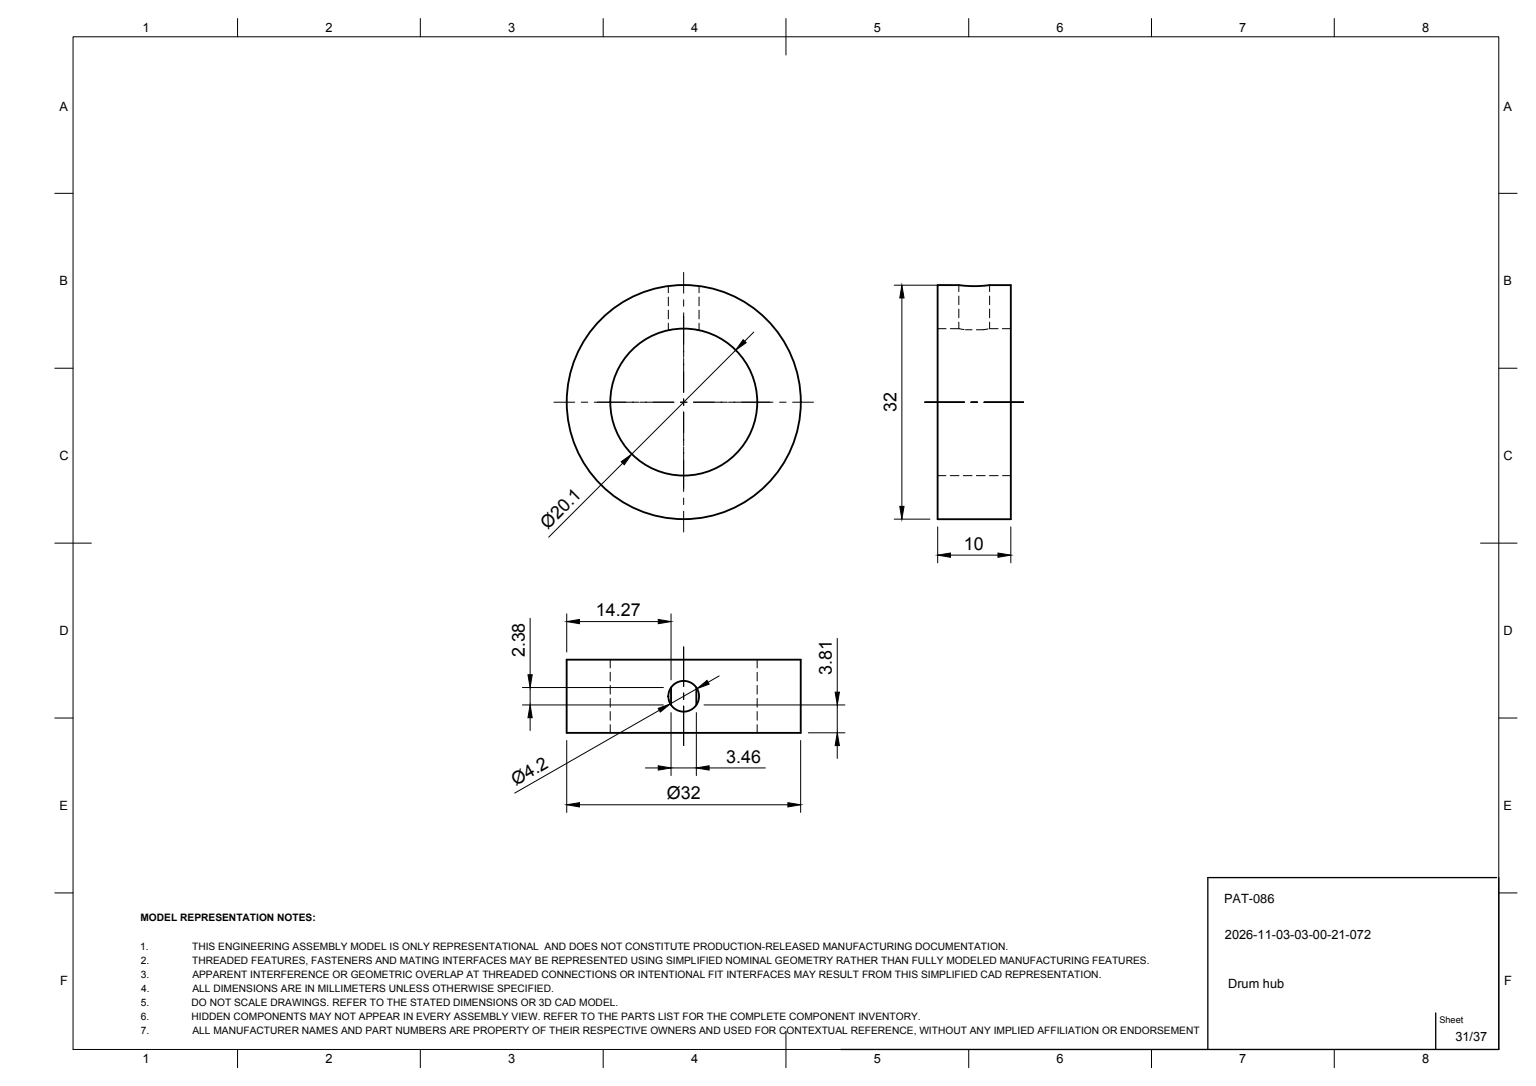
ISO-10303-21;
HEADER;
/* Generated by software containing ST-Developer
 * from STEP Tools, Inc. (www.steptools.com) 
 */

FILE_DESCRIPTION(
/* description */ ('Ratchet and pawl hand winch drum'),
/* implementation_level */ '2;1');

FILE_NAME(
/* name */ 'Drum hub.step',
/* time_stamp */ '2026-10-27T12:42:58-07:00',
/* author */ (''),
/* organization */ (''),
/* preprocessor_version */ 'ST-DEVELOPER v20.2',
/* originating_system */ 'Autodesk Translation Framework v15.17.0.0',
/* authorisation */ '');

FILE_SCHEMA (('AUTOMOTIVE_DESIGN { 1 0 10303 214 3 1 1 }'));
ENDSEC;

DATA;
#10=MECHANICAL_DESIGN_GEOMETRIC_PRESENTATION_REPRESENTATION('',(#415),#11801);
#305=B_SPLINE_CURVE_WITH_KNOTS('',3,(#10818,#10819,#10820,#10821,#10822,
#10823,#10824,#10825,#10826,#10827,#10828,#10829,#10830,#10831),
 .UNSPECIFIED.,.F.,.F.,(4,2,2,2,2,2,4),(0.756005737987019,0.793568827564647,
0.872922520054201,0.952276212543756,1.03162990503331,1.11098359752287,1.14854668710049),
 .UNSPECIFIED.);
#306=B_SPLINE_CURVE_WITH_KNOTS('',3,(#10837,#10838,#10839,#10840,#10841,
#10842,#10843,#10844,#10845,#10846,#10847,#10848,#10849,#10850,#10851,#10852,
#10853,#10854),.UNSPECIFIED.,.F.,.F.,(4,2,2,2,2,2,2,2,4),(0.,0.0792028026112439,
0.158405605222488,0.237607602356377,0.316809599490267,0.396011596624156,
0.475213593758045,0.554416396369289,0.633619198980533),.UNSPECIFIED.);
#307=B_SPLINE_CURVE_WITH_KNOTS('',3,(#10855,#10856,#10857,#10858,#10859,
#10860,#10861,#10862,#10863,#10864,#10865,#10866,#10867,#10868,#10869,#10870,
#10871,#10872),.UNSPECIFIED.,.F.,.F.,(4,2,2,2,2,2,2,2,4),(0.633619198980533,
0.712822001591777,0.792024804203021,0.87122680133691,0.950428798470799,
1.02963079560469,1.10883279273858,1.18803559534982,1.26723839796107),
 .UNSPECIFIED.);
#308=B_SPLINE_CURVE_WITH_KNOTS('',3,(#10875,#10876,#10877,#10878,#10879,
#10880,#10881,#10882,#10883,#10884,#10885,#10886,#10887,#10888),
 .UNSPECIFIED.,.F.,.F.,(4,2,2,2,2,2,4),(0.121154929624516,0.158718019202143,
0.238071711691697,0.317425404181252,0.396779096670807,0.476132789160362,
0.513695878737988),.UNSPECIFIED.);
#346=SHAPE_REPRESENTATION_RELATIONSHIP('SRR','None',#11974,#380);
#380=ADVANCED_BREP_SHAPE_REPRESENTATION('',(#448),#11791);
#415=STYLED_ITEM('',(#12199),#448);
#448=MANIFOLD_SOLID_BREP('Body1',#6294);
#576=FACE_BOUND('',#1548,.T.);
#577=FACE_BOUND('',#1550,.T.);
#578=FACE_BOUND('',#1552,.T.);
#579=FACE_BOUND('',#1554,.T.);
#740=PLANE('',#7105);
#741=PLANE('',#7110);
#742=PLANE('',#7117);
#743=PLANE('',#7118);
#1068=FACE_OUTER_BOUND('',#1544,.T.);
#1069=FACE_OUTER_BOUND('',#1545,.T.);
#1070=FACE_OUTER_BOUND('',#1546,.T.);
#1071=FACE_OUTER_BOUND('',#1547,.T.);
#1072=FACE_OUTER_BOUND('',#1549,.T.);
#1073=FACE_OUTER_BOUND('',#1551,.T.);
#1074=FACE_OUTER_BOUND('',#1553,.T.);
#1544=EDGE_LOOP('',(#5195,#5196));
#1545=EDGE_LOOP('',(#5197,#5198,#5199,#5200,#5201,#5202,#5203,#5204,#5205));
#1546=EDGE_LOOP('',(#5206,#5207,#5208));
#1547=EDGE_LOOP('',(#5209,#5210,#5211,#5212));
#1548=EDGE_LOOP('',(#5213,#5214,#5215,#5216));
#1549=EDGE_LOOP('',(#5217,#5218,#5219,#5220));
#1550=EDGE_LOOP('',(#5221,#5222));
#1551=EDGE_LOOP('',(#5223));
#1552=EDGE_LOOP('',(#5224));
#1553=EDGE_LOOP('',(#5225));
#1554=EDGE_LOOP('',(#5226));
#1973=LINE('',#10814,#2484);
#1974=LINE('',#10835,#2485);
#1975=LINE('',#10890,#2486);
#1976=LINE('',#10895,#2487);
#1977=LINE('',#10901,#2488);
#2484=VECTOR('',#8488,1.);
#2485=VECTOR('',#8495,0.21);
#2486=VECTOR('',#8500,1.);
#2487=VECTOR('',#8505,1.005);
#2488=VECTOR('',#8512,1.6);
#2885=CIRCLE('',#7106,0.21);
#2886=CIRCLE('',#7108,0.21);
#2887=CIRCLE('',#7109,0.21);
#2888=CIRCLE('',#7112,1.005);
#2889=CIRCLE('',#7113,1.005);
#2890=CIRCLE('',#7115,1.6);
#2891=CIRCLE('',#7116,1.6);
#3264=VERTEX_POINT('',#10812);
#3265=VERTEX_POINT('',#10813);
#3266=VERTEX_POINT('',#10817);
#3267=VERTEX_POINT('',#10832);
#3268=VERTEX_POINT('',#10834);
#3269=VERTEX_POINT('',#10836);
#3270=VERTEX_POINT('',#10873);
#3271=VERTEX_POINT('',#10892);
#3272=VERTEX_POINT('',#10894);
#3273=VERTEX_POINT('',#10898);
#3274=VERTEX_POINT('',#10900);
#3941=EDGE_CURVE('',#3264,#3265,#1973,.T.);
#3942=EDGE_CURVE('',#3264,#3265,#2885,.T.);
#3943=EDGE_CURVE('',#3266,#3264,#305,.T.);
#3944=EDGE_CURVE('',#3267,#3266,#2886,.T.);
#3945=EDGE_CURVE('',#3267,#3268,#1974,.T.);
#3946=EDGE_CURVE('',#3269,#3268,#306,.T.);
#3947=EDGE_CURVE('',#3268,#3269,#307,.T.);
#3948=EDGE_CURVE('',#3270,#3267,#2887,.T.);
#3949=EDGE_CURVE('',#3265,#3270,#308,.T.);
#3950=EDGE_CURVE('',#3270,#3266,#1975,.T.);
#3951=EDGE_CURVE('',#3271,#3271,#2888,.T.);
#3952=EDGE_CURVE('',#3271,#3272,#1976,.T.);
#3953=EDGE_CURVE('',#3272,#3272,#2889,.T.);
#3954=EDGE_CURVE('',#3273,#3273,#2890,.T.);
#3955=EDGE_CURVE('',#3273,#3274,#1977,.T.);
#3956=EDGE_CURVE('',#3274,#3274,#2891,.T.);
#5195=ORIENTED_EDGE('',*,*,#3941,.F.);
#5196=ORIENTED_EDGE('',*,*,#3942,.T.);
#5197=ORIENTED_EDGE('',*,*,#3943,.F.);
#5198=ORIENTED_EDGE('',*,*,#3944,.F.);
#5199=ORIENTED_EDGE('',*,*,#3945,.T.);
#5200=ORIENTED_EDGE('',*,*,#3946,.F.);
#5201=ORIENTED_EDGE('',*,*,#3947,.F.);
#5202=ORIENTED_EDGE('',*,*,#3945,.F.);
#5203=ORIENTED_EDGE('',*,*,#3948,.F.);
#5204=ORIENTED_EDGE('',*,*,#3949,.F.);
#5205=ORIENTED_EDGE('',*,*,#3942,.F.);
#5206=ORIENTED_EDGE('',*,*,#3950,.F.);
#5207=ORIENTED_EDGE('',*,*,#3948,.T.);
#5208=ORIENTED_EDGE('',*,*,#3944,.T.);
#5209=ORIENTED_EDGE('',*,*,#3951,.F.);
#5210=ORIENTED_EDGE('',*,*,#3952,.T.);
#5211=ORIENTED_EDGE('',*,*,#3953,.T.);
#5212=ORIENTED_EDGE('',*,*,#3952,.F.);
#5213=ORIENTED_EDGE('',*,*,#3949,.T.);
#5214=ORIENTED_EDGE('',*,*,#3950,.T.);
#5215=ORIENTED_EDGE('',*,*,#3943,.T.);
#5216=ORIENTED_EDGE('',*,*,#3941,.T.);
#5217=ORIENTED_EDGE('',*,*,#3954,.F.);
#5218=ORIENTED_EDGE('',*,*,#3955,.T.);
#5219=ORIENTED_EDGE('',*,*,#3956,.T.);
#5220=ORIENTED_EDGE('',*,*,#3955,.F.);
#5221=ORIENTED_EDGE('',*,*,#3946,.T.);
#5222=ORIENTED_EDGE('',*,*,#3947,.T.);
#5223=ORIENTED_EDGE('',*,*,#3954,.T.);
#5224=ORIENTED_EDGE('',*,*,#3951,.T.);
#5225=ORIENTED_EDGE('',*,*,#3956,.F.);
#5226=ORIENTED_EDGE('',*,*,#3953,.F.);
#5888=CYLINDRICAL_SURFACE('',#7107,0.21);
#5889=CYLINDRICAL_SURFACE('',#7111,1.005);
#5890=CYLINDRICAL_SURFACE('',#7114,1.6);
#6138=ADVANCED_FACE('',(#1068),#740,.T.);
#6139=ADVANCED_FACE('',(#1069),#5888,.F.);
#6140=ADVANCED_FACE('',(#1070),#741,.T.);
#6141=ADVANCED_FACE('',(#1071,#576),#5889,.F.);
#6142=ADVANCED_FACE('',(#1072,#577),#5890,.T.);
#6143=ADVANCED_FACE('',(#1073,#578),#742,.T.);
#6144=ADVANCED_FACE('',(#1074,#579),#743,.F.);
#6294=CLOSED_SHELL('',(#6138,#6139,#6140,#6141,#6142,#6143,#6144));
#7104=AXIS2_PLACEMENT_3D('',#10810,#8484,#8485);
#7105=AXIS2_PLACEMENT_3D('',#10811,#8486,#8487);
#7106=AXIS2_PLACEMENT_3D('',#10815,#8489,#8490);
#7107=AXIS2_PLACEMENT_3D('',#10816,#8491,#8492);
#7108=AXIS2_PLACEMENT_3D('',#10833,#8493,#8494);
#7109=AXIS2_PLACEMENT_3D('',#10874,#8496,#8497);
#7110=AXIS2_PLACEMENT_3D('',#10889,#8498,#8499);
#7111=AXIS2_PLACEMENT_3D('',#10891,#8501,#8502);
#7112=AXIS2_PLACEMENT_3D('',#10893,#8503,#8504);
#7113=AXIS2_PLACEMENT_3D('',#10896,#8506,#8507);
#7114=AXIS2_PLACEMENT_3D('',#10897,#8508,#8509);
#7115=AXIS2_PLACEMENT_3D('',#10899,#8510,#8511);
#7116=AXIS2_PLACEMENT_3D('',#10902,#8513,#8514);
#7117=AXIS2_PLACEMENT_3D('',#10903,#8515,#8516);
#7118=AXIS2_PLACEMENT_3D('',#10904,#8517,#8518);
#8484=DIRECTION('axis',(0.,0.,1.));
#8485=DIRECTION('refdir',(1.,0.,0.));
#8486=DIRECTION('center_axis',(0.,0.,1.));
#8487=DIRECTION('ref_axis',(1.,0.,0.));
#8488=DIRECTION('',(0.,1.,0.));
#8489=DIRECTION('center_axis',(0.,0.,1.));
#8490=DIRECTION('ref_axis',(1.,0.,0.));
#8491=DIRECTION('center_axis',(0.,0.,1.));
#8492=DIRECTION('ref_axis',(1.,0.,0.));
#8493=DIRECTION('center_axis',(0.,0.,1.));
#8494=DIRECTION('ref_axis',(1.,0.,0.));
#8495=DIRECTION('',(0.,0.,1.));
#8496=DIRECTION('center_axis',(0.,0.,1.));
#8497=DIRECTION('ref_axis',(1.,0.,0.));
#8498=DIRECTION('center_axis',(0.,0.,1.));
#8499=DIRECTION('ref_axis',(1.,0.,0.));
#8500=DIRECTION('',(0.,-1.,0.));
#8501=DIRECTION('center_axis',(0.,1.,0.));
#8502=DIRECTION('ref_axis',(1.,0.,0.));
#8503=DIRECTION('center_axis',(0.,-1.,0.));
#8504=DIRECTION('ref_axis',(1.,0.,0.));
#8505=DIRECTION('',(0.,-1.,0.));
#8506=DIRECTION('center_axis',(0.,-1.,0.));
#8507=DIRECTION('ref_axis',(1.,0.,0.));
#8508=DIRECTION('center_axis',(0.,1.,0.));
#8509=DIRECTION('ref_axis',(1.,0.,0.));
#8510=DIRECTION('center_axis',(0.,1.,0.));
#8511=DIRECTION('ref_axis',(1.,0.,0.));
#8512=DIRECTION('',(0.,-1.,0.));
#8513=DIRECTION('center_axis',(0.,1.,0.));
#8514=DIRECTION('ref_axis',(1.,0.,0.));
#8515=DIRECTION('center_axis',(0.,1.,0.));
#8516=DIRECTION('ref_axis',(1.,0.,0.));
#8517=DIRECTION('center_axis',(0.,1.,0.));
#8518=DIRECTION('ref_axis',(1.,0.,0.));
#10810=CARTESIAN_POINT('',(0.,0.,0.));
#10811=CARTESIAN_POINT('Origin',(0.,3.5,7.52));
#10812=CARTESIAN_POINT('',(0.172988438920056,3.38094119100209,7.52));
#10813=CARTESIAN_POINT('',(0.172988438920056,3.61905880899792,7.52));
#10814=CARTESIAN_POINT('',(0.172988438920056,3.,7.52));
#10815=CARTESIAN_POINT('Origin',(0.,3.5,7.52));
#10816=CARTESIAN_POINT('Origin',(0.,3.5,7.52));
#10817=CARTESIAN_POINT('',(-0.172988438920056,3.38094119100209,7.52));
#10818=CARTESIAN_POINT('Ctrl Pts',(-0.172988438920056,3.38094119100209,
7.52));
#10819=CARTESIAN_POINT('Ctrl Pts',(-0.165594865311315,3.37019857760471,
7.52129192197638));
#10820=CARTESIAN_POINT('Ctrl Pts',(-0.157297138725606,3.36031229062726,
7.52265394943905));
#10821=CARTESIAN_POINT('Ctrl Pts',(-0.129892073845076,3.33290722574673,
7.5267480843909));
#10822=CARTESIAN_POINT('Ctrl Pts',(-0.106330167759285,3.31675794366705,
7.52969589327638));
#10823=CARTESIAN_POINT('Ctrl Pts',(-0.0546129046324106,3.29530220603509,
7.53385029472357));
#10824=CARTESIAN_POINT('Ctrl Pts',(-0.0264512308298517,3.29,7.535));
#10825=CARTESIAN_POINT('Ctrl Pts',(0.0264512308298516,3.29,7.535));
#10826=CARTESIAN_POINT('Ctrl Pts',(0.0546129046324105,3.29530220603509,
7.53385029472357));
#10827=CARTESIAN_POINT('Ctrl Pts',(0.106330167759284,3.31675794366705,7.52969589327638));
#10828=CARTESIAN_POINT('Ctrl Pts',(0.129892073845076,3.33290722574673,7.5267480843909));
#10829=CARTESIAN_POINT('Ctrl Pts',(0.157297138725606,3.36031229062726,7.52265394943905));
#10830=CARTESIAN_POINT('Ctrl Pts',(0.165594865311315,3.37019857760471,7.52129192197638));
#10831=CARTESIAN_POINT('Ctrl Pts',(0.172988438920056,3.38094119100209,7.52));
#10832=CARTESIAN_POINT('',(-0.21,3.5,7.52));
#10833=CARTESIAN_POINT('Origin',(0.,3.5,7.52));
#10834=CARTESIAN_POINT('',(-0.21,3.5,8.11615888233178));
#10835=CARTESIAN_POINT('',(-0.21,3.5,7.52));
#10836=CARTESIAN_POINT('',(0.21,3.5,8.11615888233178));
#10837=CARTESIAN_POINT('Ctrl Pts',(0.21,3.5,8.11615888233178));
#10838=CARTESIAN_POINT('Ctrl Pts',(0.21,3.47359906579625,8.11615888233178));
#10839=CARTESIAN_POINT('Ctrl Pts',(0.20471752266132,3.44545944463489,8.11688606295397));
#10840=CARTESIAN_POINT('Ctrl Pts',(0.183276841782292,3.3937289476995,8.11950502964782));
#10841=CARTESIAN_POINT('Ctrl Pts',(0.167120287247804,3.37013543914945,8.12135816887013));
#10842=CARTESIAN_POINT('Ctrl Pts',(0.129864750292352,3.332879902194,8.12483075953278));
#10843=CARTESIAN_POINT('Ctrl Pts',(0.106271159541076,3.31672319916877,8.12667690933009));
#10844=CARTESIAN_POINT('Ctrl Pts',(0.0545403836274688,3.2952824096556,8.12927985626981));
#10845=CARTESIAN_POINT('Ctrl Pts',(0.0264006657112965,3.29,8.13));
#10846=CARTESIAN_POINT('Ctrl Pts',(-0.0264006657112964,3.29,8.13));
#10847=CARTESIAN_POINT('Ctrl Pts',(-0.0545403836274688,3.2952824096556,
8.12927985626981));
#10848=CARTESIAN_POINT('Ctrl Pts',(-0.106271159541076,3.31672319916877,
8.12667690933009));
#10849=CARTESIAN_POINT('Ctrl Pts',(-0.129864750292352,3.332879902194,8.12483075953278));
#10850=CARTESIAN_POINT('Ctrl Pts',(-0.167120287247804,3.37013543914945,
8.12135816887013));
#10851=CARTESIAN_POINT('Ctrl Pts',(-0.183276841782292,3.3937289476995,8.11950502964782));
#10852=CARTESIAN_POINT('Ctrl Pts',(-0.20471752266132,3.44545944463489,8.11688606295397));
#10853=CARTESIAN_POINT('Ctrl Pts',(-0.21,3.47359906579625,8.11615888233178));
#10854=CARTESIAN_POINT('Ctrl Pts',(-0.21,3.5,8.11615888233178));
#10855=CARTESIAN_POINT('Ctrl Pts',(-0.21,3.5,8.11615888233178));
#10856=CARTESIAN_POINT('Ctrl Pts',(-0.21,3.52640093420375,8.11615888233178));
#10857=CARTESIAN_POINT('Ctrl Pts',(-0.20471752266132,3.55454055536511,8.11688606295397));
#10858=CARTESIAN_POINT('Ctrl Pts',(-0.183276841782292,3.6062710523005,8.11950502964782));
#10859=CARTESIAN_POINT('Ctrl Pts',(-0.167120287247804,3.62986456085055,
8.12135816887013));
#10860=CARTESIAN_POINT('Ctrl Pts',(-0.129864750292352,3.667120097806,8.12483075953278));
#10861=CARTESIAN_POINT('Ctrl Pts',(-0.106271159541076,3.68327680083123,
8.12667690933009));
#10862=CARTESIAN_POINT('Ctrl Pts',(-0.0545403836274688,3.7047175903444,
8.12927985626981));
#10863=CARTESIAN_POINT('Ctrl Pts',(-0.0264006657112965,3.71,8.13));
#10864=CARTESIAN_POINT('Ctrl Pts',(0.0264006657112965,3.71,8.13));
#10865=CARTESIAN_POINT('Ctrl Pts',(0.0545403836274689,3.7047175903444,8.12927985626981));
#10866=CARTESIAN_POINT('Ctrl Pts',(0.106271159541076,3.68327680083123,8.12667690933009));
#10867=CARTESIAN_POINT('Ctrl Pts',(0.129864750292352,3.667120097806,8.12483075953278));
#10868=CARTESIAN_POINT('Ctrl Pts',(0.167120287247804,3.62986456085055,8.12135816887013));
#10869=CARTESIAN_POINT('Ctrl Pts',(0.183276841782292,3.6062710523005,8.11950502964782));
#10870=CARTESIAN_POINT('Ctrl Pts',(0.20471752266132,3.55454055536511,8.11688606295397));
#10871=CARTESIAN_POINT('Ctrl Pts',(0.21,3.52640093420375,8.11615888233178));
#10872=CARTESIAN_POINT('Ctrl Pts',(0.21,3.5,8.11615888233178));
#10873=CARTESIAN_POINT('',(-0.172988438920056,3.61905880899792,7.52));
#10874=CARTESIAN_POINT('Origin',(0.,3.5,7.52));
#10875=CARTESIAN_POINT('Ctrl Pts',(0.172988438920056,3.61905880899792,7.52));
#10876=CARTESIAN_POINT('Ctrl Pts',(0.165594865311314,3.62980142239529,7.52129192197638));
#10877=CARTESIAN_POINT('Ctrl Pts',(0.157297138725606,3.63968770937274,7.52265394943905));
#10878=CARTESIAN_POINT('Ctrl Pts',(0.129892073845076,3.66709277425327,7.5267480843909));
#10879=CARTESIAN_POINT('Ctrl Pts',(0.106330167759284,3.68324205633295,7.52969589327638));
#10880=CARTESIAN_POINT('Ctrl Pts',(0.0546129046324106,3.70469779396491,
7.53385029472357));
#10881=CARTESIAN_POINT('Ctrl Pts',(0.0264512308298516,3.71,7.535));
#10882=CARTESIAN_POINT('Ctrl Pts',(-0.0264512308298516,3.71,7.535));
#10883=CARTESIAN_POINT('Ctrl Pts',(-0.0546129046324105,3.70469779396491,
7.53385029472357));
#10884=CARTESIAN_POINT('Ctrl Pts',(-0.106330167759284,3.68324205633295,
7.52969589327638));
#10885=CARTESIAN_POINT('Ctrl Pts',(-0.129892073845076,3.66709277425327,
7.5267480843909));
#10886=CARTESIAN_POINT('Ctrl Pts',(-0.157297138725606,3.63968770937274,
7.52265394943905));
#10887=CARTESIAN_POINT('Ctrl Pts',(-0.165594865311314,3.62980142239529,
7.52129192197638));
#10888=CARTESIAN_POINT('Ctrl Pts',(-0.172988438920056,3.61905880899792,
7.52));
#10889=CARTESIAN_POINT('Origin',(0.,3.5,7.52));
#10890=CARTESIAN_POINT('',(-0.172988438920056,3.,7.52));
#10891=CARTESIAN_POINT('Origin',(0.,3.,6.53));
#10892=CARTESIAN_POINT('',(-1.005,4.,6.53));
#10893=CARTESIAN_POINT('Origin',(0.,4.,6.53));
#10894=CARTESIAN_POINT('',(-1.005,3.,6.53));
#10895=CARTESIAN_POINT('',(-1.005,3.,6.53));
#10896=CARTESIAN_POINT('Origin',(0.,3.,6.53));
#10897=CARTESIAN_POINT('Origin',(0.,3.,6.53));
#10898=CARTESIAN_POINT('',(-1.6,4.,6.53));
#10899=CARTESIAN_POINT('Origin',(0.,4.,6.53));
#10900=CARTESIAN_POINT('',(-1.6,3.,6.53));
#10901=CARTESIAN_POINT('',(-1.6,3.,6.53));
#10902=CARTESIAN_POINT('Origin',(0.,3.,6.53));
#10903=CARTESIAN_POINT('Origin',(0.,4.,6.53));
#10904=CARTESIAN_POINT('Origin',(0.,3.,6.53));
#11751=UNCERTAINTY_MEASURE_WITH_UNIT(LENGTH_MEASURE(0.001),#11802,
'DISTANCE_ACCURACY_VALUE',
'Maximum model space distance between geometric entities at asserted c
onnectivities');
#11761=UNCERTAINTY_MEASURE_WITH_UNIT(LENGTH_MEASURE(0.001),#11802,
'DISTANCE_ACCURACY_VALUE',
'Maximum model space distance between geometric entities at asserted c
onnectivities');
#11791=(
GEOMETRIC_REPRESENTATION_CONTEXT(3)
GLOBAL_UNCERTAINTY_ASSIGNED_CONTEXT((#11751))
GLOBAL_UNIT_ASSIGNED_CONTEXT((#11802,#11804,#11805))
REPRESENTATION_CONTEXT('','3D')
);
#11801=(
GEOMETRIC_REPRESENTATION_CONTEXT(3)
GLOBAL_UNCERTAINTY_ASSIGNED_CONTEXT((#11761))
GLOBAL_UNIT_ASSIGNED_CONTEXT((#11802,#11804,#11805))
REPRESENTATION_CONTEXT('','3D')
);
#11802=(
LENGTH_UNIT()
NAMED_UNIT(*)
SI_UNIT(.CENTI.,.METRE.)
);
#11804=(
NAMED_UNIT(*)
PLANE_ANGLE_UNIT()
SI_UNIT($,.RADIAN.)
);
#11805=(
NAMED_UNIT(*)
SI_UNIT($,.STERADIAN.)
SOLID_ANGLE_UNIT()
);
#11835=SHAPE_DEFINITION_REPRESENTATION(#11876,#11974);
#11876=PRODUCT_DEFINITION_SHAPE('',$,#12014);
#11974=SHAPE_REPRESENTATION('',(#7104),#11791);
#11984=PRODUCT_DEFINITION_CONTEXT('part definition',#12103,'design');
#12014=PRODUCT_DEFINITION('Drum hub','Drum hub',#12053,#11984);
#12053=PRODUCT_DEFINITION_FORMATION('',$,#12134);
#12103=APPLICATION_CONTEXT(
'Core Data for Automotive Mechanical Design Process');
#12104=PRODUCT_CONTEXT('part definition',#12103,'mechanical');
#12134=PRODUCT('Drum hub','Drum hub','Drum hub',(#12104));
#12193=COLOUR_RGB('Light Blue',0.38,0.62,0.78);
#12194=FILL_AREA_STYLE_COLOUR('',#12193);
#12195=FILL_AREA_STYLE('',(#12194));
#12196=SURFACE_STYLE_FILL_AREA(#12195);
#12197=SURFACE_SIDE_STYLE('',(#12196));
#12198=SURFACE_STYLE_USAGE(.BOTH.,#12197);
#12199=PRESENTATION_STYLE_ASSIGNMENT((#12198));
ENDSEC;
END-ISO-10303-21;
